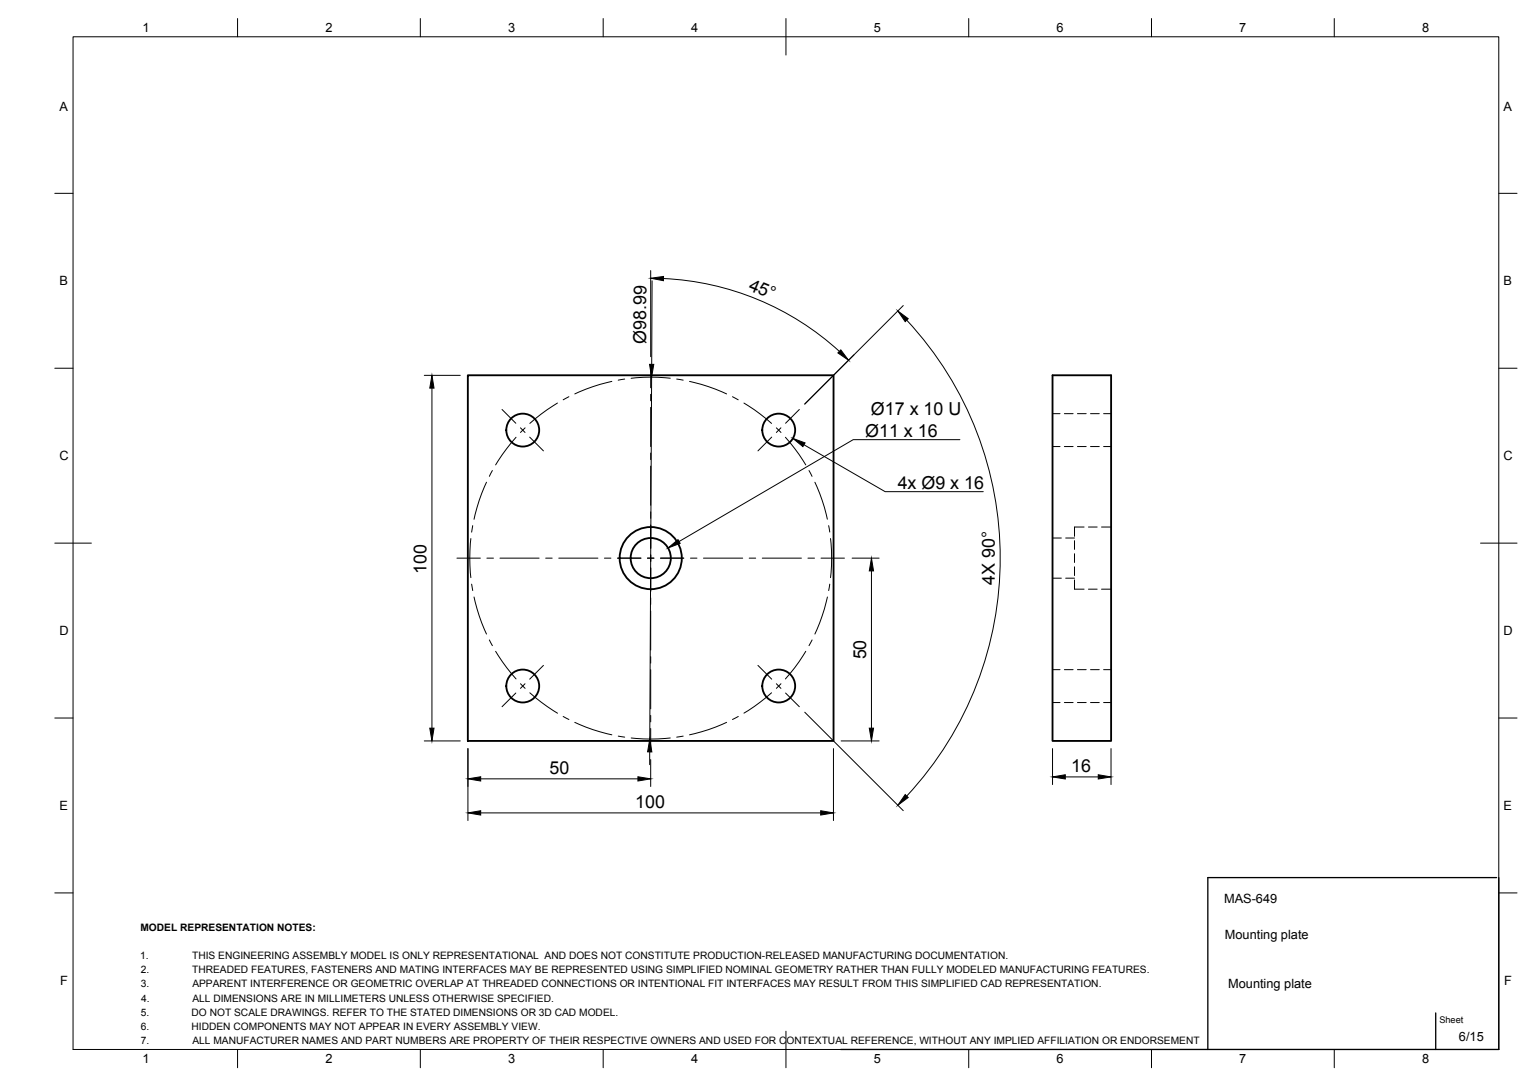
ISO-10303-21;
HEADER;
/* Generated by software containing ST-Developer
 * from STEP Tools, Inc. (www.steptools.com) 
 */

FILE_DESCRIPTION(
/* description */ ('Independent equipment support assembly with bolted 600 x 500 mm welde
d perimeter frame, four adjustable legs and swivel feet. Nominal overa
ll height 518 mm. No load rating assigned.'),
/* implementation_level */ '2;1');

FILE_NAME(
/* name */ 'Mounting plate.step',
/* time_stamp */ '2026-11-07T17:30:39-08:00',
/* author */ (''),
/* organization */ (''),
/* preprocessor_version */ 'ST-DEVELOPER v20.2',
/* originating_system */ 'Autodesk Translation Framework v15.17.0.0',
/* authorisation */ '');

FILE_SCHEMA (('AUTOMOTIVE_DESIGN { 1 0 10303 214 3 1 1 }'));
ENDSEC;

DATA;
#10=MECHANICAL_DESIGN_GEOMETRIC_PRESENTATION_REPRESENTATION('',(#2214),#63755);
#406=CIRCLE('',#15055,8.5);
#407=CIRCLE('',#15056,5.5);
#408=CIRCLE('',#15058,8.5);
#409=CIRCLE('',#15060,5.5);
#410=CIRCLE('',#15062,4.5);
#411=CIRCLE('',#15063,4.5);
#412=CIRCLE('',#15065,4.5);
#413=CIRCLE('',#15066,4.5);
#414=CIRCLE('',#15068,4.5);
#415=CIRCLE('',#15069,4.5);
#416=CIRCLE('',#15071,4.5);
#417=CIRCLE('',#15072,4.5);
#1890=CYLINDRICAL_SURFACE('',#15057,8.5);
#1891=CYLINDRICAL_SURFACE('',#15059,5.5);
#1892=CYLINDRICAL_SURFACE('',#15061,4.5);
#1893=CYLINDRICAL_SURFACE('',#15064,4.5);
#1894=CYLINDRICAL_SURFACE('',#15067,4.5);
#1895=CYLINDRICAL_SURFACE('',#15070,4.5);
#2182=SHAPE_REPRESENTATION_RELATIONSHIP('SRR','None',#63867,#2198);
#2198=ADVANCED_BREP_SHAPE_REPRESENTATION('',(#2230),#63745);
#2214=STYLED_ITEM('',(#63962),#2230);
#2230=MANIFOLD_SOLID_BREP('Body1',#14315);
#2268=FACE_BOUND('',#3487,.T.);
#2269=FACE_BOUND('',#3499,.T.);
#2270=FACE_BOUND('',#3500,.T.);
#2271=FACE_BOUND('',#3501,.T.);
#2272=FACE_BOUND('',#3502,.T.);
#2273=FACE_BOUND('',#3503,.T.);
#2274=FACE_BOUND('',#3505,.T.);
#2275=FACE_BOUND('',#3506,.T.);
#2276=FACE_BOUND('',#3507,.T.);
#2277=FACE_BOUND('',#3508,.T.);
#2278=FACE_BOUND('',#3509,.T.);
#2698=FACE_OUTER_BOUND('',#3486,.T.);
#2699=FACE_OUTER_BOUND('',#3488,.T.);
#2700=FACE_OUTER_BOUND('',#3489,.T.);
#2701=FACE_OUTER_BOUND('',#3490,.T.);
#2702=FACE_OUTER_BOUND('',#3491,.T.);
#2703=FACE_OUTER_BOUND('',#3492,.T.);
#2704=FACE_OUTER_BOUND('',#3493,.T.);
#2705=FACE_OUTER_BOUND('',#3494,.T.);
#2706=FACE_OUTER_BOUND('',#3495,.T.);
#2707=FACE_OUTER_BOUND('',#3496,.T.);
#2708=FACE_OUTER_BOUND('',#3497,.T.);
#2709=FACE_OUTER_BOUND('',#3498,.T.);
#2710=FACE_OUTER_BOUND('',#3504,.T.);
#3486=EDGE_LOOP('',(#11401));
#3487=EDGE_LOOP('',(#11402));
#3488=EDGE_LOOP('',(#11403,#11404,#11405,#11406));
#3489=EDGE_LOOP('',(#11407,#11408,#11409,#11410));
#3490=EDGE_LOOP('',(#11411,#11412,#11413,#11414));
#3491=EDGE_LOOP('',(#11415,#11416,#11417,#11418));
#3492=EDGE_LOOP('',(#11419,#11420,#11421,#11422));
#3493=EDGE_LOOP('',(#11423,#11424,#11425,#11426));
#3494=EDGE_LOOP('',(#11427,#11428,#11429,#11430));
#3495=EDGE_LOOP('',(#11431,#11432,#11433,#11434));
#3496=EDGE_LOOP('',(#11435,#11436,#11437,#11438));
#3497=EDGE_LOOP('',(#11439,#11440,#11441,#11442));
#3498=EDGE_LOOP('',(#11443,#11444,#11445,#11446));
#3499=EDGE_LOOP('',(#11447));
#3500=EDGE_LOOP('',(#11448));
#3501=EDGE_LOOP('',(#11449));
#3502=EDGE_LOOP('',(#11450));
#3503=EDGE_LOOP('',(#11451));
#3504=EDGE_LOOP('',(#11452,#11453,#11454,#11455));
#3505=EDGE_LOOP('',(#11456));
#3506=EDGE_LOOP('',(#11457));
#3507=EDGE_LOOP('',(#11458));
#3508=EDGE_LOOP('',(#11459));
#3509=EDGE_LOOP('',(#11460));
#4361=LINE('',#43976,#5197);
#4362=LINE('',#43979,#5198);
#4363=LINE('',#43985,#5199);
#4364=LINE('',#43991,#5200);
#4365=LINE('',#43997,#5201);
#4366=LINE('',#44003,#5202);
#4367=LINE('',#44008,#5203);
#4368=LINE('',#44010,#5204);
#4369=LINE('',#44012,#5205);
#4370=LINE('',#44013,#5206);
#4371=LINE('',#44016,#5207);
#4372=LINE('',#44018,#5208);
#4373=LINE('',#44019,#5209);
#4374=LINE('',#44022,#5210);
#4375=LINE('',#44024,#5211);
#4376=LINE('',#44025,#5212);
#4377=LINE('',#44027,#5213);
#4378=LINE('',#44028,#5214);
#5197=VECTOR('',#17104,8.5);
#5198=VECTOR('',#17107,5.5);
#5199=VECTOR('',#17114,4.5);
#5200=VECTOR('',#17121,4.5);
#5201=VECTOR('',#17128,4.5);
#5202=VECTOR('',#17135,4.5);
#5203=VECTOR('',#17140,10.);
#5204=VECTOR('',#17141,10.);
#5205=VECTOR('',#17142,10.);
#5206=VECTOR('',#17143,10.);
#5207=VECTOR('',#17146,10.);
#5208=VECTOR('',#17147,10.);
#5209=VECTOR('',#17148,10.);
#5210=VECTOR('',#17151,10.);
#5211=VECTOR('',#17152,10.);
#5212=VECTOR('',#17153,10.);
#5213=VECTOR('',#17156,10.);
#5214=VECTOR('',#17157,10.);
#6316=VERTEX_POINT('',#43969);
#6317=VERTEX_POINT('',#43971);
#6318=VERTEX_POINT('',#43974);
#6319=VERTEX_POINT('',#43978);
#6320=VERTEX_POINT('',#43982);
#6321=VERTEX_POINT('',#43984);
#6322=VERTEX_POINT('',#43988);
#6323=VERTEX_POINT('',#43990);
#6324=VERTEX_POINT('',#43994);
#6325=VERTEX_POINT('',#43996);
#6326=VERTEX_POINT('',#44000);
#6327=VERTEX_POINT('',#44002);
#6328=VERTEX_POINT('',#44006);
#6329=VERTEX_POINT('',#44007);
#6330=VERTEX_POINT('',#44009);
#6331=VERTEX_POINT('',#44011);
#6332=VERTEX_POINT('',#44015);
#6333=VERTEX_POINT('',#44017);
#6334=VERTEX_POINT('',#44021);
#6335=VERTEX_POINT('',#44023);
#8123=EDGE_CURVE('',#6316,#6316,#406,.T.);
#8124=EDGE_CURVE('',#6317,#6317,#407,.T.);
#8125=EDGE_CURVE('',#6318,#6318,#408,.T.);
#8126=EDGE_CURVE('',#6318,#6316,#4361,.T.);
#8127=EDGE_CURVE('',#6317,#6319,#4362,.T.);
#8128=EDGE_CURVE('',#6319,#6319,#409,.T.);
#8129=EDGE_CURVE('',#6320,#6320,#410,.T.);
#8130=EDGE_CURVE('',#6320,#6321,#4363,.T.);
#8131=EDGE_CURVE('',#6321,#6321,#411,.T.);
#8132=EDGE_CURVE('',#6322,#6322,#412,.T.);
#8133=EDGE_CURVE('',#6322,#6323,#4364,.T.);
#8134=EDGE_CURVE('',#6323,#6323,#413,.T.);
#8135=EDGE_CURVE('',#6324,#6324,#414,.T.);
#8136=EDGE_CURVE('',#6324,#6325,#4365,.T.);
#8137=EDGE_CURVE('',#6325,#6325,#415,.T.);
#8138=EDGE_CURVE('',#6326,#6326,#416,.T.);
#8139=EDGE_CURVE('',#6326,#6327,#4366,.T.);
#8140=EDGE_CURVE('',#6327,#6327,#417,.T.);
#8141=EDGE_CURVE('',#6328,#6329,#4367,.T.);
#8142=EDGE_CURVE('',#6329,#6330,#4368,.T.);
#8143=EDGE_CURVE('',#6331,#6330,#4369,.T.);
#8144=EDGE_CURVE('',#6328,#6331,#4370,.T.);
#8145=EDGE_CURVE('',#6332,#6328,#4371,.T.);
#8146=EDGE_CURVE('',#6333,#6331,#4372,.T.);
#8147=EDGE_CURVE('',#6332,#6333,#4373,.T.);
#8148=EDGE_CURVE('',#6334,#6332,#4374,.T.);
#8149=EDGE_CURVE('',#6335,#6333,#4375,.T.);
#8150=EDGE_CURVE('',#6334,#6335,#4376,.T.);
#8151=EDGE_CURVE('',#6329,#6334,#4377,.T.);
#8152=EDGE_CURVE('',#6330,#6335,#4378,.T.);
#11401=ORIENTED_EDGE('',*,*,#8123,.F.);
#11402=ORIENTED_EDGE('',*,*,#8124,.T.);
#11403=ORIENTED_EDGE('',*,*,#8125,.F.);
#11404=ORIENTED_EDGE('',*,*,#8126,.T.);
#11405=ORIENTED_EDGE('',*,*,#8123,.T.);
#11406=ORIENTED_EDGE('',*,*,#8126,.F.);
#11407=ORIENTED_EDGE('',*,*,#8124,.F.);
#11408=ORIENTED_EDGE('',*,*,#8127,.T.);
#11409=ORIENTED_EDGE('',*,*,#8128,.F.);
#11410=ORIENTED_EDGE('',*,*,#8127,.F.);
#11411=ORIENTED_EDGE('',*,*,#8129,.F.);
#11412=ORIENTED_EDGE('',*,*,#8130,.T.);
#11413=ORIENTED_EDGE('',*,*,#8131,.F.);
#11414=ORIENTED_EDGE('',*,*,#8130,.F.);
#11415=ORIENTED_EDGE('',*,*,#8132,.F.);
#11416=ORIENTED_EDGE('',*,*,#8133,.T.);
#11417=ORIENTED_EDGE('',*,*,#8134,.F.);
#11418=ORIENTED_EDGE('',*,*,#8133,.F.);
#11419=ORIENTED_EDGE('',*,*,#8135,.F.);
#11420=ORIENTED_EDGE('',*,*,#8136,.T.);
#11421=ORIENTED_EDGE('',*,*,#8137,.F.);
#11422=ORIENTED_EDGE('',*,*,#8136,.F.);
#11423=ORIENTED_EDGE('',*,*,#8138,.F.);
#11424=ORIENTED_EDGE('',*,*,#8139,.T.);
#11425=ORIENTED_EDGE('',*,*,#8140,.F.);
#11426=ORIENTED_EDGE('',*,*,#8139,.F.);
#11427=ORIENTED_EDGE('',*,*,#8141,.T.);
#11428=ORIENTED_EDGE('',*,*,#8142,.T.);
#11429=ORIENTED_EDGE('',*,*,#8143,.F.);
#11430=ORIENTED_EDGE('',*,*,#8144,.F.);
#11431=ORIENTED_EDGE('',*,*,#8145,.T.);
#11432=ORIENTED_EDGE('',*,*,#8144,.T.);
#11433=ORIENTED_EDGE('',*,*,#8146,.F.);
#11434=ORIENTED_EDGE('',*,*,#8147,.F.);
#11435=ORIENTED_EDGE('',*,*,#8148,.T.);
#11436=ORIENTED_EDGE('',*,*,#8147,.T.);
#11437=ORIENTED_EDGE('',*,*,#8149,.F.);
#11438=ORIENTED_EDGE('',*,*,#8150,.F.);
#11439=ORIENTED_EDGE('',*,*,#8151,.T.);
#11440=ORIENTED_EDGE('',*,*,#8150,.T.);
#11441=ORIENTED_EDGE('',*,*,#8152,.F.);
#11442=ORIENTED_EDGE('',*,*,#8142,.F.);
#11443=ORIENTED_EDGE('',*,*,#8152,.T.);
#11444=ORIENTED_EDGE('',*,*,#8149,.T.);
#11445=ORIENTED_EDGE('',*,*,#8146,.T.);
#11446=ORIENTED_EDGE('',*,*,#8143,.T.);
#11447=ORIENTED_EDGE('',*,*,#8125,.T.);
#11448=ORIENTED_EDGE('',*,*,#8129,.T.);
#11449=ORIENTED_EDGE('',*,*,#8132,.T.);
#11450=ORIENTED_EDGE('',*,*,#8135,.T.);
#11451=ORIENTED_EDGE('',*,*,#8138,.T.);
#11452=ORIENTED_EDGE('',*,*,#8151,.F.);
#11453=ORIENTED_EDGE('',*,*,#8141,.F.);
#11454=ORIENTED_EDGE('',*,*,#8145,.F.);
#11455=ORIENTED_EDGE('',*,*,#8148,.F.);
#11456=ORIENTED_EDGE('',*,*,#8128,.T.);
#11457=ORIENTED_EDGE('',*,*,#8131,.T.);
#11458=ORIENTED_EDGE('',*,*,#8134,.T.);
#11459=ORIENTED_EDGE('',*,*,#8137,.T.);
#11460=ORIENTED_EDGE('',*,*,#8140,.T.);
#13489=PLANE('',#15054);
#13490=PLANE('',#15073);
#13491=PLANE('',#15074);
#13492=PLANE('',#15075);
#13493=PLANE('',#15076);
#13494=PLANE('',#15077);
#13495=PLANE('',#15078);
#13944=ADVANCED_FACE('',(#2698,#2268),#13489,.F.);
#13945=ADVANCED_FACE('',(#2699),#1890,.F.);
#13946=ADVANCED_FACE('',(#2700),#1891,.F.);
#13947=ADVANCED_FACE('',(#2701),#1892,.F.);
#13948=ADVANCED_FACE('',(#2702),#1893,.F.);
#13949=ADVANCED_FACE('',(#2703),#1894,.F.);
#13950=ADVANCED_FACE('',(#2704),#1895,.F.);
#13951=ADVANCED_FACE('',(#2705),#13490,.T.);
#13952=ADVANCED_FACE('',(#2706),#13491,.T.);
#13953=ADVANCED_FACE('',(#2707),#13492,.T.);
#13954=ADVANCED_FACE('',(#2708),#13493,.T.);
#13955=ADVANCED_FACE('',(#2709,#2269,#2270,#2271,#2272,#2273),#13494,.T.);
#13956=ADVANCED_FACE('',(#2710,#2274,#2275,#2276,#2277,#2278),#13495,.F.);
#14315=CLOSED_SHELL('',(#13944,#13945,#13946,#13947,#13948,#13949,#13950,
#13951,#13952,#13953,#13954,#13955,#13956));
#15053=AXIS2_PLACEMENT_3D('',#43967,#17092,#17093);
#15054=AXIS2_PLACEMENT_3D('',#43968,#17094,#17095);
#15055=AXIS2_PLACEMENT_3D('',#43970,#17096,#17097);
#15056=AXIS2_PLACEMENT_3D('',#43972,#17098,#17099);
#15057=AXIS2_PLACEMENT_3D('',#43973,#17100,#17101);
#15058=AXIS2_PLACEMENT_3D('',#43975,#17102,#17103);
#15059=AXIS2_PLACEMENT_3D('',#43977,#17105,#17106);
#15060=AXIS2_PLACEMENT_3D('',#43980,#17108,#17109);
#15061=AXIS2_PLACEMENT_3D('',#43981,#17110,#17111);
#15062=AXIS2_PLACEMENT_3D('',#43983,#17112,#17113);
#15063=AXIS2_PLACEMENT_3D('',#43986,#17115,#17116);
#15064=AXIS2_PLACEMENT_3D('',#43987,#17117,#17118);
#15065=AXIS2_PLACEMENT_3D('',#43989,#17119,#17120);
#15066=AXIS2_PLACEMENT_3D('',#43992,#17122,#17123);
#15067=AXIS2_PLACEMENT_3D('',#43993,#17124,#17125);
#15068=AXIS2_PLACEMENT_3D('',#43995,#17126,#17127);
#15069=AXIS2_PLACEMENT_3D('',#43998,#17129,#17130);
#15070=AXIS2_PLACEMENT_3D('',#43999,#17131,#17132);
#15071=AXIS2_PLACEMENT_3D('',#44001,#17133,#17134);
#15072=AXIS2_PLACEMENT_3D('',#44004,#17136,#17137);
#15073=AXIS2_PLACEMENT_3D('',#44005,#17138,#17139);
#15074=AXIS2_PLACEMENT_3D('',#44014,#17144,#17145);
#15075=AXIS2_PLACEMENT_3D('',#44020,#17149,#17150);
#15076=AXIS2_PLACEMENT_3D('',#44026,#17154,#17155);
#15077=AXIS2_PLACEMENT_3D('',#44029,#17158,#17159);
#15078=AXIS2_PLACEMENT_3D('',#44030,#17160,#17161);
#17092=DIRECTION('axis',(0.,0.,1.));
#17093=DIRECTION('refdir',(1.,0.,0.));
#17094=DIRECTION('center_axis',(0.,0.,-1.));
#17095=DIRECTION('ref_axis',(1.,0.,0.));
#17096=DIRECTION('center_axis',(0.,0.,-1.));
#17097=DIRECTION('ref_axis',(1.,0.,0.));
#17098=DIRECTION('center_axis',(0.,0.,-1.));
#17099=DIRECTION('ref_axis',(1.,0.,0.));
#17100=DIRECTION('center_axis',(0.,0.,-1.));
#17101=DIRECTION('ref_axis',(1.,0.,0.));
#17102=DIRECTION('center_axis',(0.,0.,-1.));
#17103=DIRECTION('ref_axis',(1.,0.,0.));
#17104=DIRECTION('',(0.,0.,-1.));
#17105=DIRECTION('center_axis',(0.,0.,-1.));
#17106=DIRECTION('ref_axis',(1.,0.,0.));
#17107=DIRECTION('',(0.,0.,-1.));
#17108=DIRECTION('center_axis',(0.,0.,1.));
#17109=DIRECTION('ref_axis',(1.,0.,0.));
#17110=DIRECTION('center_axis',(0.,0.,-1.));
#17111=DIRECTION('ref_axis',(1.,0.,0.));
#17112=DIRECTION('center_axis',(0.,0.,-1.));
#17113=DIRECTION('ref_axis',(1.,0.,0.));
#17114=DIRECTION('',(0.,0.,-1.));
#17115=DIRECTION('center_axis',(0.,0.,1.));
#17116=DIRECTION('ref_axis',(1.,0.,0.));
#17117=DIRECTION('center_axis',(0.,0.,-1.));
#17118=DIRECTION('ref_axis',(1.,0.,0.));
#17119=DIRECTION('center_axis',(0.,0.,-1.));
#17120=DIRECTION('ref_axis',(1.,0.,0.));
#17121=DIRECTION('',(0.,0.,-1.));
#17122=DIRECTION('center_axis',(0.,0.,1.));
#17123=DIRECTION('ref_axis',(1.,0.,0.));
#17124=DIRECTION('center_axis',(0.,0.,-1.));
#17125=DIRECTION('ref_axis',(1.,0.,0.));
#17126=DIRECTION('center_axis',(0.,0.,-1.));
#17127=DIRECTION('ref_axis',(1.,0.,0.));
#17128=DIRECTION('',(0.,0.,-1.));
#17129=DIRECTION('center_axis',(0.,0.,1.));
#17130=DIRECTION('ref_axis',(1.,0.,0.));
#17131=DIRECTION('center_axis',(0.,0.,-1.));
#17132=DIRECTION('ref_axis',(1.,0.,0.));
#17133=DIRECTION('center_axis',(0.,0.,-1.));
#17134=DIRECTION('ref_axis',(1.,0.,0.));
#17135=DIRECTION('',(0.,0.,-1.));
#17136=DIRECTION('center_axis',(0.,0.,1.));
#17137=DIRECTION('ref_axis',(1.,0.,0.));
#17138=DIRECTION('center_axis',(0.,1.,0.));
#17139=DIRECTION('ref_axis',(-1.,0.,0.));
#17140=DIRECTION('',(-1.,0.,0.));
#17141=DIRECTION('',(0.,0.,1.));
#17142=DIRECTION('',(-1.,0.,0.));
#17143=DIRECTION('',(0.,0.,1.));
#17144=DIRECTION('center_axis',(1.,0.,0.));
#17145=DIRECTION('ref_axis',(0.,1.,0.));
#17146=DIRECTION('',(0.,1.,0.));
#17147=DIRECTION('',(0.,1.,0.));
#17148=DIRECTION('',(0.,0.,1.));
#17149=DIRECTION('center_axis',(0.,-1.,0.));
#17150=DIRECTION('ref_axis',(1.,0.,0.));
#17151=DIRECTION('',(1.,0.,0.));
#17152=DIRECTION('',(1.,0.,0.));
#17153=DIRECTION('',(0.,0.,1.));
#17154=DIRECTION('center_axis',(-1.,0.,0.));
#17155=DIRECTION('ref_axis',(0.,-1.,0.));
#17156=DIRECTION('',(0.,-1.,0.));
#17157=DIRECTION('',(0.,-1.,0.));
#17158=DIRECTION('center_axis',(0.,0.,1.));
#17159=DIRECTION('ref_axis',(1.,0.,0.));
#17160=DIRECTION('center_axis',(0.,0.,1.));
#17161=DIRECTION('ref_axis',(1.,0.,0.));
#43967=CARTESIAN_POINT('',(0.,0.,0.));
#43968=CARTESIAN_POINT('Origin',(0.,0.,6.));
#43969=CARTESIAN_POINT('',(-8.5,1.04094977927525E-15,6.));
#43970=CARTESIAN_POINT('Origin',(0.,0.,6.));
#43971=CARTESIAN_POINT('',(-5.5,6.73555739531044E-16,6.));
#43972=CARTESIAN_POINT('Origin',(0.,0.,6.));
#43973=CARTESIAN_POINT('Origin',(0.,0.,11.));
#43974=CARTESIAN_POINT('',(-8.5,1.04094977927525E-15,16.));
#43975=CARTESIAN_POINT('Origin',(0.,0.,16.));
#43976=CARTESIAN_POINT('',(-8.5,1.04094977927525E-15,11.));
#43977=CARTESIAN_POINT('Origin',(0.,0.,8.));
#43978=CARTESIAN_POINT('',(-5.5,6.73555739531044E-16,0.));
#43979=CARTESIAN_POINT('',(-5.5,6.73555739531044E-16,8.));
#43980=CARTESIAN_POINT('Origin',(0.,0.,0.));
#43981=CARTESIAN_POINT('Origin',(35.,-35.,8.));
#43982=CARTESIAN_POINT('',(30.5,-35.,16.));
#43983=CARTESIAN_POINT('Origin',(35.,-35.,16.));
#43984=CARTESIAN_POINT('',(30.5,-35.,0.));
#43985=CARTESIAN_POINT('',(30.5,-35.,8.));
#43986=CARTESIAN_POINT('Origin',(35.,-35.,0.));
#43987=CARTESIAN_POINT('Origin',(-35.,-35.,8.));
#43988=CARTESIAN_POINT('',(-39.5,-35.,16.));
#43989=CARTESIAN_POINT('Origin',(-35.,-35.,16.));
#43990=CARTESIAN_POINT('',(-39.5,-35.,0.));
#43991=CARTESIAN_POINT('',(-39.5,-35.,8.));
#43992=CARTESIAN_POINT('Origin',(-35.,-35.,0.));
#43993=CARTESIAN_POINT('Origin',(-35.,35.,8.));
#43994=CARTESIAN_POINT('',(-39.5,35.,16.));
#43995=CARTESIAN_POINT('Origin',(-35.,35.,16.));
#43996=CARTESIAN_POINT('',(-39.5,35.,0.));
#43997=CARTESIAN_POINT('',(-39.5,35.,8.));
#43998=CARTESIAN_POINT('Origin',(-35.,35.,0.));
#43999=CARTESIAN_POINT('Origin',(35.,35.,8.));
#44000=CARTESIAN_POINT('',(30.5,35.,16.));
#44001=CARTESIAN_POINT('Origin',(35.,35.,16.));
#44002=CARTESIAN_POINT('',(30.5,35.,0.));
#44003=CARTESIAN_POINT('',(30.5,35.,8.));
#44004=CARTESIAN_POINT('Origin',(35.,35.,0.));
#44005=CARTESIAN_POINT('Origin',(50.,50.,0.));
#44006=CARTESIAN_POINT('',(50.,50.,0.));
#44007=CARTESIAN_POINT('',(-50.,50.,0.));
#44008=CARTESIAN_POINT('',(50.,50.,0.));
#44009=CARTESIAN_POINT('',(-50.,50.,16.));
#44010=CARTESIAN_POINT('',(-50.,50.,0.));
#44011=CARTESIAN_POINT('',(50.,50.,16.));
#44012=CARTESIAN_POINT('',(50.,50.,16.));
#44013=CARTESIAN_POINT('',(50.,50.,0.));
#44014=CARTESIAN_POINT('Origin',(50.,-50.,0.));
#44015=CARTESIAN_POINT('',(50.,-50.,0.));
#44016=CARTESIAN_POINT('',(50.,-50.,0.));
#44017=CARTESIAN_POINT('',(50.,-50.,16.));
#44018=CARTESIAN_POINT('',(50.,-50.,16.));
#44019=CARTESIAN_POINT('',(50.,-50.,0.));
#44020=CARTESIAN_POINT('Origin',(-50.,-50.,0.));
#44021=CARTESIAN_POINT('',(-50.,-50.,0.));
#44022=CARTESIAN_POINT('',(-50.,-50.,0.));
#44023=CARTESIAN_POINT('',(-50.,-50.,16.));
#44024=CARTESIAN_POINT('',(-50.,-50.,16.));
#44025=CARTESIAN_POINT('',(-50.,-50.,0.));
#44026=CARTESIAN_POINT('Origin',(-50.,50.,0.));
#44027=CARTESIAN_POINT('',(-50.,50.,0.));
#44028=CARTESIAN_POINT('',(-50.,50.,16.));
#44029=CARTESIAN_POINT('Origin',(0.,0.,16.));
#44030=CARTESIAN_POINT('Origin',(0.,0.,0.));
#63725=UNCERTAINTY_MEASURE_WITH_UNIT(LENGTH_MEASURE(0.01),#63756,
'DISTANCE_ACCURACY_VALUE',
'Maximum model space distance between geometric entities at asserted c
onnectivities');
#63735=UNCERTAINTY_MEASURE_WITH_UNIT(LENGTH_MEASURE(0.01),#63756,
'DISTANCE_ACCURACY_VALUE',
'Maximum model space distance between geometric entities at asserted c
onnectivities');
#63745=(
GEOMETRIC_REPRESENTATION_CONTEXT(3)
GLOBAL_UNCERTAINTY_ASSIGNED_CONTEXT((#63725))
GLOBAL_UNIT_ASSIGNED_CONTEXT((#63756,#63758,#63759))
REPRESENTATION_CONTEXT('','3D')
);
#63755=(
GEOMETRIC_REPRESENTATION_CONTEXT(3)
GLOBAL_UNCERTAINTY_ASSIGNED_CONTEXT((#63735))
GLOBAL_UNIT_ASSIGNED_CONTEXT((#63756,#63758,#63759))
REPRESENTATION_CONTEXT('','3D')
);
#63756=(
LENGTH_UNIT()
NAMED_UNIT(*)
SI_UNIT(.MILLI.,.METRE.)
);
#63758=(
NAMED_UNIT(*)
PLANE_ANGLE_UNIT()
SI_UNIT($,.RADIAN.)
);
#63759=(
NAMED_UNIT(*)
SI_UNIT($,.STERADIAN.)
SOLID_ANGLE_UNIT()
);
#63769=SHAPE_DEFINITION_REPRESENTATION(#63828,#63867);
#63828=PRODUCT_DEFINITION_SHAPE('',$,#63887);
#63867=SHAPE_REPRESENTATION('',(#15053),#63745);
#63877=PRODUCT_DEFINITION_CONTEXT('part definition',#63936,'design');
#63887=PRODUCT_DEFINITION('Mounting plate','Mounting plate',#63906,#63877);
#63906=PRODUCT_DEFINITION_FORMATION('',$,#63947);
#63936=APPLICATION_CONTEXT(
'Core Data for Automotive Mechanical Design Process');
#63937=PRODUCT_CONTEXT('part definition',#63936,'mechanical');
#63947=PRODUCT('Mounting plate','Mounting plate','Mounting plate',(#63937));
#63962=PRESENTATION_STYLE_ASSIGNMENT((#63969));
#63969=SURFACE_STYLE_USAGE(.BOTH.,#63976);
#63976=SURFACE_SIDE_STYLE('',(#63983));
#63983=SURFACE_STYLE_FILL_AREA(#63990);
#63990=FILL_AREA_STYLE('Gray',(#63997));
#63997=FILL_AREA_STYLE_COLOUR('Gray',#64004);
#64004=COLOUR_RGB('Gray',0.407843137254902,0.447058823529412,0.498039215686275);
ENDSEC;
END-ISO-10303-21;
